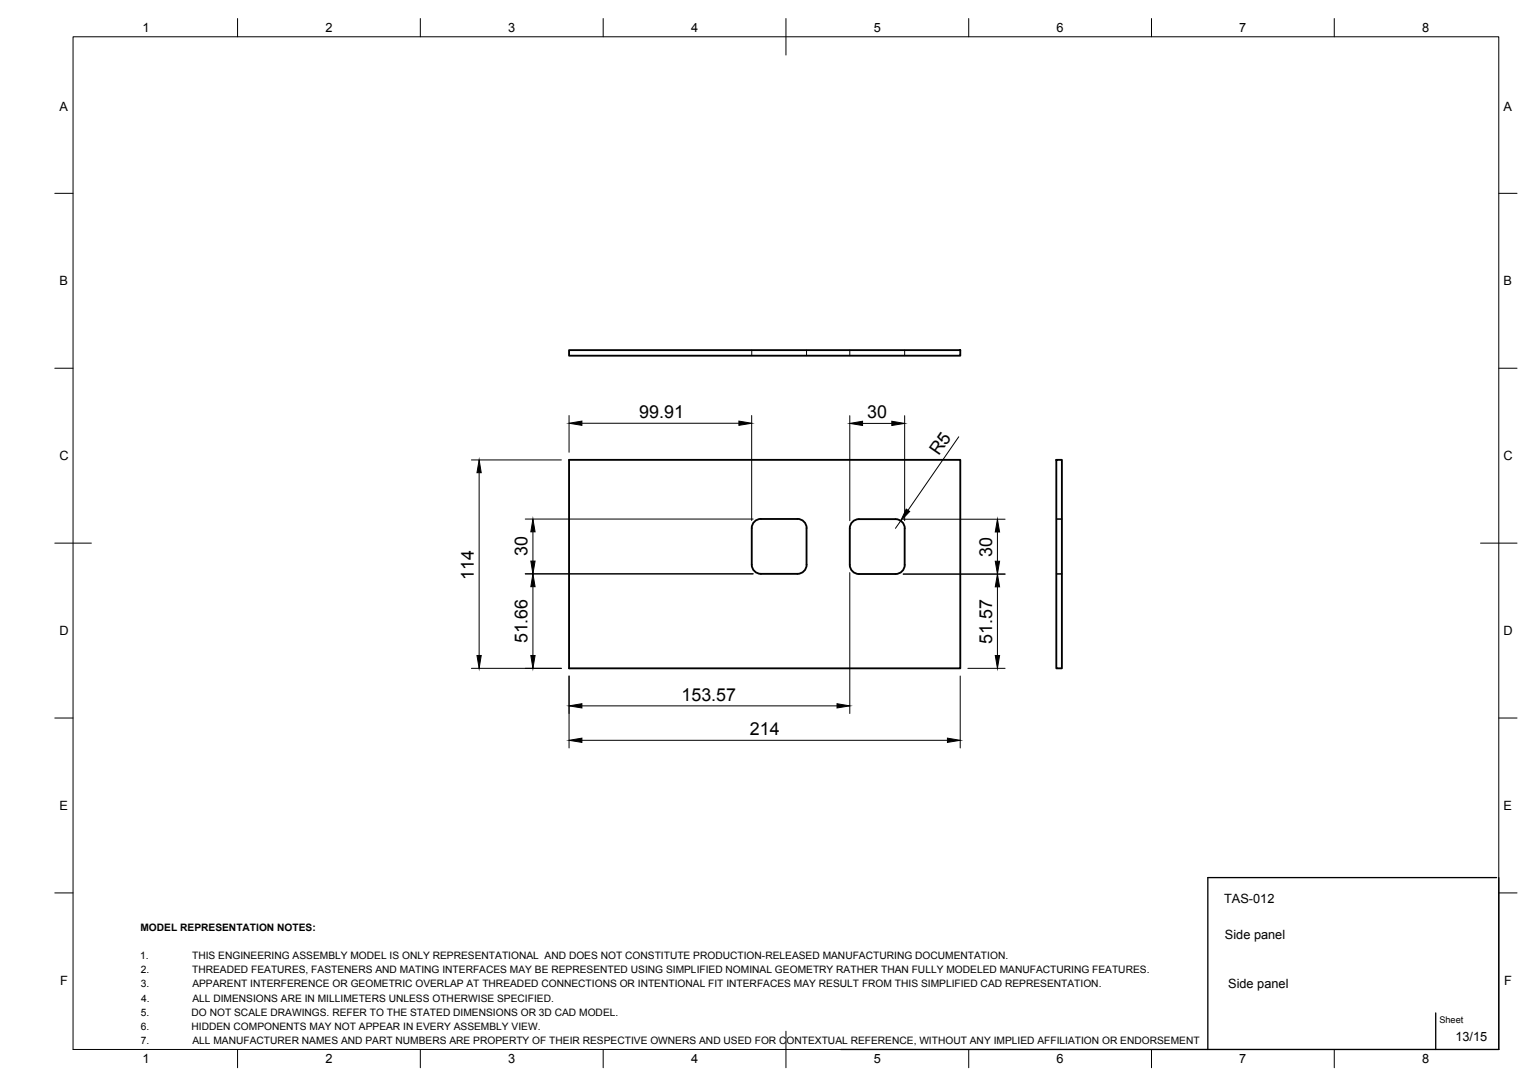
ISO-10303-21;
HEADER;
/* Generated by software containing ST-Developer
 * from STEP Tools, Inc. (www.steptools.com) 
 */

FILE_DESCRIPTION(
/* description */ (
'Independent welded steel electronics enclosure with removable sealed 
lid, internal mounting tray and two threaded cable entries. 300 x 220 
mm body. No ingress or electrical safety rating assigned.'),
/* implementation_level */ '2;1');

FILE_NAME(
/* name */ 'Side panel.step',
/* time_stamp */ '2026-11-14T09:13:27-08:00',
/* author */ (''),
/* organization */ (''),
/* preprocessor_version */ 'ST-DEVELOPER v20.2',
/* originating_system */ 'Autodesk Translation Framework v15.17.0.0',
/* authorisation */ '');

FILE_SCHEMA (('AUTOMOTIVE_DESIGN { 1 0 10303 214 3 1 1 }'));
ENDSEC;

DATA;
#10=MECHANICAL_DESIGN_GEOMETRIC_PRESENTATION_REPRESENTATION('',(#969),#94412);
#939=SHAPE_REPRESENTATION_RELATIONSHIP('SRR','None',#94491,#954);
#954=ADVANCED_BREP_SHAPE_REPRESENTATION('',(#984),#94400);
#969=STYLED_ITEM('',(#94576),#984);
#984=MANIFOLD_SOLID_BREP('Body1',#8254);
#1008=FACE_BOUND('',#1568,.T.);
#1009=FACE_BOUND('',#1569,.T.);
#1010=FACE_BOUND('',#1572,.T.);
#1011=FACE_BOUND('',#1573,.T.);
#1076=PLANE('',#8477);
#1077=PLANE('',#8481);
#1078=PLANE('',#8485);
#1079=PLANE('',#8489);
#1080=PLANE('',#8493);
#1081=PLANE('',#8497);
#1082=PLANE('',#8501);
#1083=PLANE('',#8505);
#1084=PLANE('',#8506);
#1085=PLANE('',#8507);
#1086=PLANE('',#8508);
#1087=PLANE('',#8509);
#1088=PLANE('',#8510);
#1089=PLANE('',#8511);
#1182=FACE_OUTER_BOUND('',#1550,.T.);
#1183=FACE_OUTER_BOUND('',#1551,.T.);
#1184=FACE_OUTER_BOUND('',#1552,.T.);
#1185=FACE_OUTER_BOUND('',#1553,.T.);
#1186=FACE_OUTER_BOUND('',#1554,.T.);
#1187=FACE_OUTER_BOUND('',#1555,.T.);
#1188=FACE_OUTER_BOUND('',#1556,.T.);
#1189=FACE_OUTER_BOUND('',#1557,.T.);
#1190=FACE_OUTER_BOUND('',#1558,.T.);
#1191=FACE_OUTER_BOUND('',#1559,.T.);
#1192=FACE_OUTER_BOUND('',#1560,.T.);
#1193=FACE_OUTER_BOUND('',#1561,.T.);
#1194=FACE_OUTER_BOUND('',#1562,.T.);
#1195=FACE_OUTER_BOUND('',#1563,.T.);
#1196=FACE_OUTER_BOUND('',#1564,.T.);
#1197=FACE_OUTER_BOUND('',#1565,.T.);
#1198=FACE_OUTER_BOUND('',#1566,.T.);
#1199=FACE_OUTER_BOUND('',#1567,.T.);
#1200=FACE_OUTER_BOUND('',#1570,.T.);
#1201=FACE_OUTER_BOUND('',#1571,.T.);
#1202=FACE_OUTER_BOUND('',#1574,.T.);
#1203=FACE_OUTER_BOUND('',#1575,.T.);
#1550=EDGE_LOOP('',(#5202,#5203,#5204,#5205));
#1551=EDGE_LOOP('',(#5206,#5207,#5208,#5209));
#1552=EDGE_LOOP('',(#5210,#5211,#5212,#5213));
#1553=EDGE_LOOP('',(#5214,#5215,#5216,#5217));
#1554=EDGE_LOOP('',(#5218,#5219,#5220,#5221));
#1555=EDGE_LOOP('',(#5222,#5223,#5224,#5225));
#1556=EDGE_LOOP('',(#5226,#5227,#5228,#5229));
#1557=EDGE_LOOP('',(#5230,#5231,#5232,#5233));
#1558=EDGE_LOOP('',(#5234,#5235,#5236,#5237));
#1559=EDGE_LOOP('',(#5238,#5239,#5240,#5241));
#1560=EDGE_LOOP('',(#5242,#5243,#5244,#5245));
#1561=EDGE_LOOP('',(#5246,#5247,#5248,#5249));
#1562=EDGE_LOOP('',(#5250,#5251,#5252,#5253));
#1563=EDGE_LOOP('',(#5254,#5255,#5256,#5257));
#1564=EDGE_LOOP('',(#5258,#5259,#5260,#5261));
#1565=EDGE_LOOP('',(#5262,#5263,#5264,#5265));
#1566=EDGE_LOOP('',(#5266,#5267,#5268,#5269));
#1567=EDGE_LOOP('',(#5270,#5271,#5272,#5273));
#1568=EDGE_LOOP('',(#5274,#5275,#5276,#5277,#5278,#5279,#5280,#5281));
#1569=EDGE_LOOP('',(#5282,#5283,#5284,#5285,#5286,#5287,#5288,#5289));
#1570=EDGE_LOOP('',(#5290,#5291,#5292,#5293));
#1571=EDGE_LOOP('',(#5294,#5295,#5296,#5297));
#1572=EDGE_LOOP('',(#5298,#5299,#5300,#5301,#5302,#5303,#5304,#5305));
#1573=EDGE_LOOP('',(#5306,#5307,#5308,#5309,#5310,#5311,#5312,#5313));
#1574=EDGE_LOOP('',(#5314,#5315,#5316,#5317));
#1575=EDGE_LOOP('',(#5318,#5319,#5320,#5321));
#1974=LINE('',#10485,#2372);
#1975=LINE('',#10488,#2373);
#1976=LINE('',#10491,#2374);
#1977=LINE('',#10493,#2375);
#1978=LINE('',#10494,#2376);
#1979=LINE('',#10499,#2377);
#1980=LINE('',#10503,#2378);
#1981=LINE('',#10505,#2379);
#1982=LINE('',#10506,#2380);
#1983=LINE('',#10512,#2381);
#1984=LINE('',#10515,#2382);
#1985=LINE('',#10517,#2383);
#1986=LINE('',#10518,#2384);
#1987=LINE('',#10523,#2385);
#1988=LINE('',#10526,#2386);
#1989=LINE('',#10527,#2387);
#1990=LINE('',#10533,#2388);
#1991=LINE('',#10536,#2389);
#1992=LINE('',#10539,#2390);
#1993=LINE('',#10541,#2391);
#1994=LINE('',#10542,#2392);
#1995=LINE('',#10548,#2393);
#1996=LINE('',#10551,#2394);
#1997=LINE('',#10553,#2395);
#1998=LINE('',#10554,#2396);
#1999=LINE('',#10559,#2397);
#2000=LINE('',#10563,#2398);
#2001=LINE('',#10565,#2399);
#2002=LINE('',#10566,#2400);
#2003=LINE('',#10571,#2401);
#2004=LINE('',#10574,#2402);
#2005=LINE('',#10575,#2403);
#2006=LINE('',#10579,#2404);
#2007=LINE('',#10581,#2405);
#2008=LINE('',#10583,#2406);
#2009=LINE('',#10584,#2407);
#2010=LINE('',#10587,#2408);
#2011=LINE('',#10589,#2409);
#2012=LINE('',#10590,#2410);
#2013=LINE('',#10593,#2411);
#2014=LINE('',#10595,#2412);
#2015=LINE('',#10596,#2413);
#2016=LINE('',#10598,#2414);
#2017=LINE('',#10599,#2415);
#2372=VECTOR('',#9072,10.);
#2373=VECTOR('',#9075,10.);
#2374=VECTOR('',#9078,10.);
#2375=VECTOR('',#9079,10.);
#2376=VECTOR('',#9080,10.);
#2377=VECTOR('',#9085,10.);
#2378=VECTOR('',#9090,10.);
#2379=VECTOR('',#9091,10.);
#2380=VECTOR('',#9092,10.);
#2381=VECTOR('',#9097,10.);
#2382=VECTOR('',#9100,10.);
#2383=VECTOR('',#9103,10.);
#2384=VECTOR('',#9104,10.);
#2385=VECTOR('',#9109,10.);
#2386=VECTOR('',#9114,10.);
#2387=VECTOR('',#9115,10.);
#2388=VECTOR('',#9120,10.);
#2389=VECTOR('',#9123,10.);
#2390=VECTOR('',#9126,10.);
#2391=VECTOR('',#9127,10.);
#2392=VECTOR('',#9128,10.);
#2393=VECTOR('',#9133,10.);
#2394=VECTOR('',#9136,10.);
#2395=VECTOR('',#9139,10.);
#2396=VECTOR('',#9140,10.);
#2397=VECTOR('',#9145,10.);
#2398=VECTOR('',#9150,10.);
#2399=VECTOR('',#9151,10.);
#2400=VECTOR('',#9152,10.);
#2401=VECTOR('',#9157,10.);
#2402=VECTOR('',#9162,10.);
#2403=VECTOR('',#9163,10.);
#2404=VECTOR('',#9166,10.);
#2405=VECTOR('',#9167,10.);
#2406=VECTOR('',#9168,10.);
#2407=VECTOR('',#9169,10.);
#2408=VECTOR('',#9172,10.);
#2409=VECTOR('',#9173,10.);
#2410=VECTOR('',#9174,10.);
#2411=VECTOR('',#9177,10.);
#2412=VECTOR('',#9178,10.);
#2413=VECTOR('',#9179,10.);
#2414=VECTOR('',#9182,10.);
#2415=VECTOR('',#9183,10.);
#2740=CIRCLE('',#8475,5.);
#2741=CIRCLE('',#8476,5.);
#2742=CIRCLE('',#8479,5.);
#2743=CIRCLE('',#8480,5.);
#2744=CIRCLE('',#8483,5.);
#2745=CIRCLE('',#8484,5.);
#2746=CIRCLE('',#8487,5.);
#2747=CIRCLE('',#8488,5.);
#2748=CIRCLE('',#8491,5.);
#2749=CIRCLE('',#8492,5.);
#2750=CIRCLE('',#8495,5.);
#2751=CIRCLE('',#8496,5.);
#2752=CIRCLE('',#8499,5.);
#2753=CIRCLE('',#8500,5.);
#2754=CIRCLE('',#8503,5.);
#2755=CIRCLE('',#8504,5.);
#2882=VERTEX_POINT('',#10481);
#2883=VERTEX_POINT('',#10482);
#2884=VERTEX_POINT('',#10484);
#2885=VERTEX_POINT('',#10486);
#2886=VERTEX_POINT('',#10490);
#2887=VERTEX_POINT('',#10492);
#2888=VERTEX_POINT('',#10496);
#2889=VERTEX_POINT('',#10498);
#2890=VERTEX_POINT('',#10502);
#2891=VERTEX_POINT('',#10504);
#2892=VERTEX_POINT('',#10508);
#2893=VERTEX_POINT('',#10509);
#2894=VERTEX_POINT('',#10511);
#2895=VERTEX_POINT('',#10513);
#2896=VERTEX_POINT('',#10520);
#2897=VERTEX_POINT('',#10522);
#2898=VERTEX_POINT('',#10529);
#2899=VERTEX_POINT('',#10530);
#2900=VERTEX_POINT('',#10532);
#2901=VERTEX_POINT('',#10534);
#2902=VERTEX_POINT('',#10538);
#2903=VERTEX_POINT('',#10540);
#2904=VERTEX_POINT('',#10544);
#2905=VERTEX_POINT('',#10545);
#2906=VERTEX_POINT('',#10547);
#2907=VERTEX_POINT('',#10549);
#2908=VERTEX_POINT('',#10556);
#2909=VERTEX_POINT('',#10558);
#2910=VERTEX_POINT('',#10562);
#2911=VERTEX_POINT('',#10564);
#2912=VERTEX_POINT('',#10568);
#2913=VERTEX_POINT('',#10570);
#2914=VERTEX_POINT('',#10577);
#2915=VERTEX_POINT('',#10578);
#2916=VERTEX_POINT('',#10580);
#2917=VERTEX_POINT('',#10582);
#2918=VERTEX_POINT('',#10586);
#2919=VERTEX_POINT('',#10588);
#2920=VERTEX_POINT('',#10592);
#2921=VERTEX_POINT('',#10594);
#3866=EDGE_CURVE('',#2882,#2883,#2740,.T.);
#3867=EDGE_CURVE('',#2883,#2884,#1974,.T.);
#3868=EDGE_CURVE('',#2884,#2885,#2741,.T.);
#3869=EDGE_CURVE('',#2885,#2882,#1975,.T.);
#3870=EDGE_CURVE('',#2886,#2883,#1976,.T.);
#3871=EDGE_CURVE('',#2887,#2886,#1977,.T.);
#3872=EDGE_CURVE('',#2884,#2887,#1978,.T.);
#3873=EDGE_CURVE('',#2886,#2888,#2742,.T.);
#3874=EDGE_CURVE('',#2888,#2889,#1979,.T.);
#3875=EDGE_CURVE('',#2889,#2887,#2743,.T.);
#3876=EDGE_CURVE('',#2890,#2888,#1980,.T.);
#3877=EDGE_CURVE('',#2891,#2890,#1981,.T.);
#3878=EDGE_CURVE('',#2889,#2891,#1982,.T.);
#3879=EDGE_CURVE('',#2892,#2893,#2744,.T.);
#3880=EDGE_CURVE('',#2893,#2894,#1983,.T.);
#3881=EDGE_CURVE('',#2894,#2895,#2745,.T.);
#3882=EDGE_CURVE('',#2895,#2892,#1984,.T.);
#3883=EDGE_CURVE('',#2894,#2885,#1985,.T.);
#3884=EDGE_CURVE('',#2882,#2893,#1986,.T.);
#3885=EDGE_CURVE('',#2890,#2896,#2746,.T.);
#3886=EDGE_CURVE('',#2896,#2897,#1987,.T.);
#3887=EDGE_CURVE('',#2897,#2891,#2747,.T.);
#3888=EDGE_CURVE('',#2897,#2895,#1988,.T.);
#3889=EDGE_CURVE('',#2892,#2896,#1989,.T.);
#3890=EDGE_CURVE('',#2898,#2899,#2748,.T.);
#3891=EDGE_CURVE('',#2899,#2900,#1990,.T.);
#3892=EDGE_CURVE('',#2900,#2901,#2749,.T.);
#3893=EDGE_CURVE('',#2901,#2898,#1991,.T.);
#3894=EDGE_CURVE('',#2902,#2899,#1992,.T.);
#3895=EDGE_CURVE('',#2903,#2902,#1993,.T.);
#3896=EDGE_CURVE('',#2900,#2903,#1994,.T.);
#3897=EDGE_CURVE('',#2904,#2905,#2750,.T.);
#3898=EDGE_CURVE('',#2905,#2906,#1995,.T.);
#3899=EDGE_CURVE('',#2906,#2907,#2751,.T.);
#3900=EDGE_CURVE('',#2907,#2904,#1996,.T.);
#3901=EDGE_CURVE('',#2906,#2901,#1997,.T.);
#3902=EDGE_CURVE('',#2898,#2905,#1998,.T.);
#3903=EDGE_CURVE('',#2902,#2908,#2752,.T.);
#3904=EDGE_CURVE('',#2908,#2909,#1999,.T.);
#3905=EDGE_CURVE('',#2909,#2903,#2753,.T.);
#3906=EDGE_CURVE('',#2910,#2908,#2000,.T.);
#3907=EDGE_CURVE('',#2911,#2910,#2001,.T.);
#3908=EDGE_CURVE('',#2909,#2911,#2002,.T.);
#3909=EDGE_CURVE('',#2910,#2912,#2754,.T.);
#3910=EDGE_CURVE('',#2912,#2913,#2003,.T.);
#3911=EDGE_CURVE('',#2913,#2911,#2755,.T.);
#3912=EDGE_CURVE('',#2913,#2907,#2004,.T.);
#3913=EDGE_CURVE('',#2904,#2912,#2005,.T.);
#3914=EDGE_CURVE('',#2914,#2915,#2006,.T.);
#3915=EDGE_CURVE('',#2915,#2916,#2007,.T.);
#3916=EDGE_CURVE('',#2917,#2916,#2008,.T.);
#3917=EDGE_CURVE('',#2914,#2917,#2009,.T.);
#3918=EDGE_CURVE('',#2918,#2914,#2010,.T.);
#3919=EDGE_CURVE('',#2919,#2917,#2011,.T.);
#3920=EDGE_CURVE('',#2918,#2919,#2012,.T.);
#3921=EDGE_CURVE('',#2920,#2918,#2013,.T.);
#3922=EDGE_CURVE('',#2921,#2919,#2014,.T.);
#3923=EDGE_CURVE('',#2920,#2921,#2015,.T.);
#3924=EDGE_CURVE('',#2915,#2920,#2016,.T.);
#3925=EDGE_CURVE('',#2916,#2921,#2017,.T.);
#5202=ORIENTED_EDGE('',*,*,#3866,.T.);
#5203=ORIENTED_EDGE('',*,*,#3867,.T.);
#5204=ORIENTED_EDGE('',*,*,#3868,.T.);
#5205=ORIENTED_EDGE('',*,*,#3869,.T.);
#5206=ORIENTED_EDGE('',*,*,#3867,.F.);
#5207=ORIENTED_EDGE('',*,*,#3870,.F.);
#5208=ORIENTED_EDGE('',*,*,#3871,.F.);
#5209=ORIENTED_EDGE('',*,*,#3872,.F.);
#5210=ORIENTED_EDGE('',*,*,#3873,.T.);
#5211=ORIENTED_EDGE('',*,*,#3874,.T.);
#5212=ORIENTED_EDGE('',*,*,#3875,.T.);
#5213=ORIENTED_EDGE('',*,*,#3871,.T.);
#5214=ORIENTED_EDGE('',*,*,#3874,.F.);
#5215=ORIENTED_EDGE('',*,*,#3876,.F.);
#5216=ORIENTED_EDGE('',*,*,#3877,.F.);
#5217=ORIENTED_EDGE('',*,*,#3878,.F.);
#5218=ORIENTED_EDGE('',*,*,#3879,.T.);
#5219=ORIENTED_EDGE('',*,*,#3880,.T.);
#5220=ORIENTED_EDGE('',*,*,#3881,.T.);
#5221=ORIENTED_EDGE('',*,*,#3882,.T.);
#5222=ORIENTED_EDGE('',*,*,#3869,.F.);
#5223=ORIENTED_EDGE('',*,*,#3883,.F.);
#5224=ORIENTED_EDGE('',*,*,#3880,.F.);
#5225=ORIENTED_EDGE('',*,*,#3884,.F.);
#5226=ORIENTED_EDGE('',*,*,#3885,.T.);
#5227=ORIENTED_EDGE('',*,*,#3886,.T.);
#5228=ORIENTED_EDGE('',*,*,#3887,.T.);
#5229=ORIENTED_EDGE('',*,*,#3877,.T.);
#5230=ORIENTED_EDGE('',*,*,#3882,.F.);
#5231=ORIENTED_EDGE('',*,*,#3888,.F.);
#5232=ORIENTED_EDGE('',*,*,#3886,.F.);
#5233=ORIENTED_EDGE('',*,*,#3889,.F.);
#5234=ORIENTED_EDGE('',*,*,#3890,.T.);
#5235=ORIENTED_EDGE('',*,*,#3891,.T.);
#5236=ORIENTED_EDGE('',*,*,#3892,.T.);
#5237=ORIENTED_EDGE('',*,*,#3893,.T.);
#5238=ORIENTED_EDGE('',*,*,#3891,.F.);
#5239=ORIENTED_EDGE('',*,*,#3894,.F.);
#5240=ORIENTED_EDGE('',*,*,#3895,.F.);
#5241=ORIENTED_EDGE('',*,*,#3896,.F.);
#5242=ORIENTED_EDGE('',*,*,#3897,.T.);
#5243=ORIENTED_EDGE('',*,*,#3898,.T.);
#5244=ORIENTED_EDGE('',*,*,#3899,.T.);
#5245=ORIENTED_EDGE('',*,*,#3900,.T.);
#5246=ORIENTED_EDGE('',*,*,#3893,.F.);
#5247=ORIENTED_EDGE('',*,*,#3901,.F.);
#5248=ORIENTED_EDGE('',*,*,#3898,.F.);
#5249=ORIENTED_EDGE('',*,*,#3902,.F.);
#5250=ORIENTED_EDGE('',*,*,#3903,.T.);
#5251=ORIENTED_EDGE('',*,*,#3904,.T.);
#5252=ORIENTED_EDGE('',*,*,#3905,.T.);
#5253=ORIENTED_EDGE('',*,*,#3895,.T.);
#5254=ORIENTED_EDGE('',*,*,#3904,.F.);
#5255=ORIENTED_EDGE('',*,*,#3906,.F.);
#5256=ORIENTED_EDGE('',*,*,#3907,.F.);
#5257=ORIENTED_EDGE('',*,*,#3908,.F.);
#5258=ORIENTED_EDGE('',*,*,#3909,.T.);
#5259=ORIENTED_EDGE('',*,*,#3910,.T.);
#5260=ORIENTED_EDGE('',*,*,#3911,.T.);
#5261=ORIENTED_EDGE('',*,*,#3907,.T.);
#5262=ORIENTED_EDGE('',*,*,#3900,.F.);
#5263=ORIENTED_EDGE('',*,*,#3912,.F.);
#5264=ORIENTED_EDGE('',*,*,#3910,.F.);
#5265=ORIENTED_EDGE('',*,*,#3913,.F.);
#5266=ORIENTED_EDGE('',*,*,#3914,.T.);
#5267=ORIENTED_EDGE('',*,*,#3915,.T.);
#5268=ORIENTED_EDGE('',*,*,#3916,.F.);
#5269=ORIENTED_EDGE('',*,*,#3917,.F.);
#5270=ORIENTED_EDGE('',*,*,#3918,.T.);
#5271=ORIENTED_EDGE('',*,*,#3917,.T.);
#5272=ORIENTED_EDGE('',*,*,#3919,.F.);
#5273=ORIENTED_EDGE('',*,*,#3920,.F.);
#5274=ORIENTED_EDGE('',*,*,#3906,.T.);
#5275=ORIENTED_EDGE('',*,*,#3903,.F.);
#5276=ORIENTED_EDGE('',*,*,#3894,.T.);
#5277=ORIENTED_EDGE('',*,*,#3890,.F.);
#5278=ORIENTED_EDGE('',*,*,#3902,.T.);
#5279=ORIENTED_EDGE('',*,*,#3897,.F.);
#5280=ORIENTED_EDGE('',*,*,#3913,.T.);
#5281=ORIENTED_EDGE('',*,*,#3909,.F.);
#5282=ORIENTED_EDGE('',*,*,#3870,.T.);
#5283=ORIENTED_EDGE('',*,*,#3866,.F.);
#5284=ORIENTED_EDGE('',*,*,#3884,.T.);
#5285=ORIENTED_EDGE('',*,*,#3879,.F.);
#5286=ORIENTED_EDGE('',*,*,#3889,.T.);
#5287=ORIENTED_EDGE('',*,*,#3885,.F.);
#5288=ORIENTED_EDGE('',*,*,#3876,.T.);
#5289=ORIENTED_EDGE('',*,*,#3873,.F.);
#5290=ORIENTED_EDGE('',*,*,#3921,.T.);
#5291=ORIENTED_EDGE('',*,*,#3920,.T.);
#5292=ORIENTED_EDGE('',*,*,#3922,.F.);
#5293=ORIENTED_EDGE('',*,*,#3923,.F.);
#5294=ORIENTED_EDGE('',*,*,#3924,.T.);
#5295=ORIENTED_EDGE('',*,*,#3923,.T.);
#5296=ORIENTED_EDGE('',*,*,#3925,.F.);
#5297=ORIENTED_EDGE('',*,*,#3915,.F.);
#5298=ORIENTED_EDGE('',*,*,#3908,.T.);
#5299=ORIENTED_EDGE('',*,*,#3911,.F.);
#5300=ORIENTED_EDGE('',*,*,#3912,.T.);
#5301=ORIENTED_EDGE('',*,*,#3899,.F.);
#5302=ORIENTED_EDGE('',*,*,#3901,.T.);
#5303=ORIENTED_EDGE('',*,*,#3892,.F.);
#5304=ORIENTED_EDGE('',*,*,#3896,.T.);
#5305=ORIENTED_EDGE('',*,*,#3905,.F.);
#5306=ORIENTED_EDGE('',*,*,#3872,.T.);
#5307=ORIENTED_EDGE('',*,*,#3875,.F.);
#5308=ORIENTED_EDGE('',*,*,#3878,.T.);
#5309=ORIENTED_EDGE('',*,*,#3887,.F.);
#5310=ORIENTED_EDGE('',*,*,#3888,.T.);
#5311=ORIENTED_EDGE('',*,*,#3881,.F.);
#5312=ORIENTED_EDGE('',*,*,#3883,.T.);
#5313=ORIENTED_EDGE('',*,*,#3868,.F.);
#5314=ORIENTED_EDGE('',*,*,#3925,.T.);
#5315=ORIENTED_EDGE('',*,*,#3922,.T.);
#5316=ORIENTED_EDGE('',*,*,#3919,.T.);
#5317=ORIENTED_EDGE('',*,*,#3916,.T.);
#5318=ORIENTED_EDGE('',*,*,#3924,.F.);
#5319=ORIENTED_EDGE('',*,*,#3914,.F.);
#5320=ORIENTED_EDGE('',*,*,#3918,.F.);
#5321=ORIENTED_EDGE('',*,*,#3921,.F.);
#7664=CYLINDRICAL_SURFACE('',#8474,5.);
#7665=CYLINDRICAL_SURFACE('',#8478,5.);
#7666=CYLINDRICAL_SURFACE('',#8482,5.);
#7667=CYLINDRICAL_SURFACE('',#8486,5.);
#7668=CYLINDRICAL_SURFACE('',#8490,5.);
#7669=CYLINDRICAL_SURFACE('',#8494,5.);
#7670=CYLINDRICAL_SURFACE('',#8498,5.);
#7671=CYLINDRICAL_SURFACE('',#8502,5.);
#7919=ADVANCED_FACE('',(#1182),#7664,.F.);
#7920=ADVANCED_FACE('',(#1183),#1076,.F.);
#7921=ADVANCED_FACE('',(#1184),#7665,.F.);
#7922=ADVANCED_FACE('',(#1185),#1077,.F.);
#7923=ADVANCED_FACE('',(#1186),#7666,.F.);
#7924=ADVANCED_FACE('',(#1187),#1078,.F.);
#7925=ADVANCED_FACE('',(#1188),#7667,.F.);
#7926=ADVANCED_FACE('',(#1189),#1079,.F.);
#7927=ADVANCED_FACE('',(#1190),#7668,.F.);
#7928=ADVANCED_FACE('',(#1191),#1080,.F.);
#7929=ADVANCED_FACE('',(#1192),#7669,.F.);
#7930=ADVANCED_FACE('',(#1193),#1081,.F.);
#7931=ADVANCED_FACE('',(#1194),#7670,.F.);
#7932=ADVANCED_FACE('',(#1195),#1082,.F.);
#7933=ADVANCED_FACE('',(#1196),#7671,.F.);
#7934=ADVANCED_FACE('',(#1197),#1083,.F.);
#7935=ADVANCED_FACE('',(#1198),#1084,.T.);
#7936=ADVANCED_FACE('',(#1199,#1008,#1009),#1085,.T.);
#7937=ADVANCED_FACE('',(#1200),#1086,.T.);
#7938=ADVANCED_FACE('',(#1201,#1010,#1011),#1087,.T.);
#7939=ADVANCED_FACE('',(#1202),#1088,.T.);
#7940=ADVANCED_FACE('',(#1203),#1089,.F.);
#8254=CLOSED_SHELL('',(#7919,#7920,#7921,#7922,#7923,#7924,#7925,#7926,
#7927,#7928,#7929,#7930,#7931,#7932,#7933,#7934,#7935,#7936,#7937,#7938,
#7939,#7940));
#8473=AXIS2_PLACEMENT_3D('',#10479,#9066,#9067);
#8474=AXIS2_PLACEMENT_3D('',#10480,#9068,#9069);
#8475=AXIS2_PLACEMENT_3D('',#10483,#9070,#9071);
#8476=AXIS2_PLACEMENT_3D('',#10487,#9073,#9074);
#8477=AXIS2_PLACEMENT_3D('',#10489,#9076,#9077);
#8478=AXIS2_PLACEMENT_3D('',#10495,#9081,#9082);
#8479=AXIS2_PLACEMENT_3D('',#10497,#9083,#9084);
#8480=AXIS2_PLACEMENT_3D('',#10500,#9086,#9087);
#8481=AXIS2_PLACEMENT_3D('',#10501,#9088,#9089);
#8482=AXIS2_PLACEMENT_3D('',#10507,#9093,#9094);
#8483=AXIS2_PLACEMENT_3D('',#10510,#9095,#9096);
#8484=AXIS2_PLACEMENT_3D('',#10514,#9098,#9099);
#8485=AXIS2_PLACEMENT_3D('',#10516,#9101,#9102);
#8486=AXIS2_PLACEMENT_3D('',#10519,#9105,#9106);
#8487=AXIS2_PLACEMENT_3D('',#10521,#9107,#9108);
#8488=AXIS2_PLACEMENT_3D('',#10524,#9110,#9111);
#8489=AXIS2_PLACEMENT_3D('',#10525,#9112,#9113);
#8490=AXIS2_PLACEMENT_3D('',#10528,#9116,#9117);
#8491=AXIS2_PLACEMENT_3D('',#10531,#9118,#9119);
#8492=AXIS2_PLACEMENT_3D('',#10535,#9121,#9122);
#8493=AXIS2_PLACEMENT_3D('',#10537,#9124,#9125);
#8494=AXIS2_PLACEMENT_3D('',#10543,#9129,#9130);
#8495=AXIS2_PLACEMENT_3D('',#10546,#9131,#9132);
#8496=AXIS2_PLACEMENT_3D('',#10550,#9134,#9135);
#8497=AXIS2_PLACEMENT_3D('',#10552,#9137,#9138);
#8498=AXIS2_PLACEMENT_3D('',#10555,#9141,#9142);
#8499=AXIS2_PLACEMENT_3D('',#10557,#9143,#9144);
#8500=AXIS2_PLACEMENT_3D('',#10560,#9146,#9147);
#8501=AXIS2_PLACEMENT_3D('',#10561,#9148,#9149);
#8502=AXIS2_PLACEMENT_3D('',#10567,#9153,#9154);
#8503=AXIS2_PLACEMENT_3D('',#10569,#9155,#9156);
#8504=AXIS2_PLACEMENT_3D('',#10572,#9158,#9159);
#8505=AXIS2_PLACEMENT_3D('',#10573,#9160,#9161);
#8506=AXIS2_PLACEMENT_3D('',#10576,#9164,#9165);
#8507=AXIS2_PLACEMENT_3D('',#10585,#9170,#9171);
#8508=AXIS2_PLACEMENT_3D('',#10591,#9175,#9176);
#8509=AXIS2_PLACEMENT_3D('',#10597,#9180,#9181);
#8510=AXIS2_PLACEMENT_3D('',#10600,#9184,#9185);
#8511=AXIS2_PLACEMENT_3D('',#10601,#9186,#9187);
#9066=DIRECTION('axis',(0.,0.,1.));
#9067=DIRECTION('refdir',(1.,0.,0.));
#9068=DIRECTION('center_axis',(-1.,0.,0.));
#9069=DIRECTION('ref_axis',(0.,-0.707106781186548,0.707106781186548));
#9070=DIRECTION('center_axis',(1.,0.,0.));
#9071=DIRECTION('ref_axis',(0.,-0.707106781186548,0.707106781186548));
#9072=DIRECTION('',(-1.,0.,0.));
#9073=DIRECTION('center_axis',(-1.,0.,0.));
#9074=DIRECTION('ref_axis',(0.,-0.707106781186548,0.707106781186548));
#9075=DIRECTION('',(1.,0.,0.));
#9076=DIRECTION('center_axis',(0.,-1.,0.));
#9077=DIRECTION('ref_axis',(0.,0.,1.));
#9078=DIRECTION('',(0.,0.,1.));
#9079=DIRECTION('',(1.,0.,0.));
#9080=DIRECTION('',(0.,0.,-1.));
#9081=DIRECTION('center_axis',(-1.,0.,0.));
#9082=DIRECTION('ref_axis',(0.,-0.707106781186548,-0.707106781186548));
#9083=DIRECTION('center_axis',(1.,0.,0.));
#9084=DIRECTION('ref_axis',(0.,-0.707106781186548,-0.707106781186548));
#9085=DIRECTION('',(-1.,0.,0.));
#9086=DIRECTION('center_axis',(-1.,0.,0.));
#9087=DIRECTION('ref_axis',(0.,-0.707106781186548,-0.707106781186548));
#9088=DIRECTION('center_axis',(0.,0.,-1.));
#9089=DIRECTION('ref_axis',(0.,-1.,0.));
#9090=DIRECTION('',(0.,-1.,0.));
#9091=DIRECTION('',(1.,0.,0.));
#9092=DIRECTION('',(0.,1.,0.));
#9093=DIRECTION('center_axis',(-1.,0.,0.));
#9094=DIRECTION('ref_axis',(0.,0.707106781186548,0.707106781186548));
#9095=DIRECTION('center_axis',(1.,0.,0.));
#9096=DIRECTION('ref_axis',(0.,0.707106781186548,0.707106781186548));
#9097=DIRECTION('',(-1.,0.,0.));
#9098=DIRECTION('center_axis',(-1.,0.,0.));
#9099=DIRECTION('ref_axis',(0.,0.707106781186548,0.707106781186548));
#9100=DIRECTION('',(1.,0.,0.));
#9101=DIRECTION('center_axis',(0.,0.,1.));
#9102=DIRECTION('ref_axis',(0.,1.,0.));
#9103=DIRECTION('',(0.,-1.,0.));
#9104=DIRECTION('',(0.,1.,0.));
#9105=DIRECTION('center_axis',(-1.,0.,0.));
#9106=DIRECTION('ref_axis',(0.,0.707106781186548,-0.707106781186548));
#9107=DIRECTION('center_axis',(1.,0.,0.));
#9108=DIRECTION('ref_axis',(0.,0.707106781186548,-0.707106781186548));
#9109=DIRECTION('',(-1.,0.,0.));
#9110=DIRECTION('center_axis',(-1.,0.,0.));
#9111=DIRECTION('ref_axis',(0.,0.707106781186548,-0.707106781186548));
#9112=DIRECTION('center_axis',(0.,1.,0.));
#9113=DIRECTION('ref_axis',(0.,0.,-1.));
#9114=DIRECTION('',(0.,0.,1.));
#9115=DIRECTION('',(0.,0.,-1.));
#9116=DIRECTION('center_axis',(-1.,0.,0.));
#9117=DIRECTION('ref_axis',(0.,0.707106781186548,0.707106781186548));
#9118=DIRECTION('center_axis',(1.,0.,0.));
#9119=DIRECTION('ref_axis',(0.,0.707106781186548,0.707106781186548));
#9120=DIRECTION('',(-1.,0.,0.));
#9121=DIRECTION('center_axis',(-1.,0.,0.));
#9122=DIRECTION('ref_axis',(0.,0.707106781186548,0.707106781186548));
#9123=DIRECTION('',(1.,0.,0.));
#9124=DIRECTION('center_axis',(0.,0.,1.));
#9125=DIRECTION('ref_axis',(0.,1.,0.));
#9126=DIRECTION('',(0.,1.,0.));
#9127=DIRECTION('',(1.,0.,0.));
#9128=DIRECTION('',(0.,-1.,0.));
#9129=DIRECTION('center_axis',(-1.,0.,0.));
#9130=DIRECTION('ref_axis',(0.,0.707106781186548,-0.707106781186548));
#9131=DIRECTION('center_axis',(1.,0.,0.));
#9132=DIRECTION('ref_axis',(0.,0.707106781186548,-0.707106781186548));
#9133=DIRECTION('',(-1.,0.,0.));
#9134=DIRECTION('center_axis',(-1.,0.,0.));
#9135=DIRECTION('ref_axis',(0.,0.707106781186548,-0.707106781186548));
#9136=DIRECTION('',(1.,0.,0.));
#9137=DIRECTION('center_axis',(0.,1.,0.));
#9138=DIRECTION('ref_axis',(0.,0.,-1.));
#9139=DIRECTION('',(0.,0.,1.));
#9140=DIRECTION('',(0.,0.,-1.));
#9141=DIRECTION('center_axis',(-1.,0.,0.));
#9142=DIRECTION('ref_axis',(0.,-0.707106781186548,0.707106781186548));
#9143=DIRECTION('center_axis',(1.,0.,0.));
#9144=DIRECTION('ref_axis',(0.,-0.707106781186548,0.707106781186548));
#9145=DIRECTION('',(-1.,0.,0.));
#9146=DIRECTION('center_axis',(-1.,0.,0.));
#9147=DIRECTION('ref_axis',(0.,-0.707106781186548,0.707106781186548));
#9148=DIRECTION('center_axis',(0.,-1.,0.));
#9149=DIRECTION('ref_axis',(0.,0.,1.));
#9150=DIRECTION('',(0.,0.,1.));
#9151=DIRECTION('',(1.,0.,0.));
#9152=DIRECTION('',(0.,0.,-1.));
#9153=DIRECTION('center_axis',(-1.,0.,0.));
#9154=DIRECTION('ref_axis',(0.,-0.707106781186548,-0.707106781186548));
#9155=DIRECTION('center_axis',(1.,0.,0.));
#9156=DIRECTION('ref_axis',(0.,-0.707106781186548,-0.707106781186548));
#9157=DIRECTION('',(-1.,0.,0.));
#9158=DIRECTION('center_axis',(-1.,0.,0.));
#9159=DIRECTION('ref_axis',(0.,-0.707106781186548,-0.707106781186548));
#9160=DIRECTION('center_axis',(0.,0.,-1.));
#9161=DIRECTION('ref_axis',(0.,-1.,0.));
#9162=DIRECTION('',(0.,1.,0.));
#9163=DIRECTION('',(0.,-1.,0.));
#9164=DIRECTION('center_axis',(0.,1.,0.));
#9165=DIRECTION('ref_axis',(-1.,0.,0.));
#9166=DIRECTION('',(-1.,0.,0.));
#9167=DIRECTION('',(0.,0.,1.));
#9168=DIRECTION('',(-1.,0.,0.));
#9169=DIRECTION('',(0.,0.,1.));
#9170=DIRECTION('center_axis',(1.,0.,0.));
#9171=DIRECTION('ref_axis',(0.,1.,0.));
#9172=DIRECTION('',(0.,1.,0.));
#9173=DIRECTION('',(0.,1.,0.));
#9174=DIRECTION('',(0.,0.,1.));
#9175=DIRECTION('center_axis',(0.,-1.,0.));
#9176=DIRECTION('ref_axis',(1.,0.,0.));
#9177=DIRECTION('',(1.,0.,0.));
#9178=DIRECTION('',(1.,0.,0.));
#9179=DIRECTION('',(0.,0.,1.));
#9180=DIRECTION('center_axis',(-1.,0.,0.));
#9181=DIRECTION('ref_axis',(0.,-1.,0.));
#9182=DIRECTION('',(0.,-1.,0.));
#9183=DIRECTION('',(0.,-1.,0.));
#9184=DIRECTION('center_axis',(0.,0.,1.));
#9185=DIRECTION('ref_axis',(1.,0.,0.));
#9186=DIRECTION('center_axis',(0.,0.,1.));
#9187=DIRECTION('ref_axis',(1.,0.,0.));
#10479=CARTESIAN_POINT('',(0.,0.,0.));
#10480=CARTESIAN_POINT('Origin',(298.5,-17.9108928257202,76.6590099406496));
#10481=CARTESIAN_POINT('',(1.5,-17.9108928257202,81.6590099406496));
#10482=CARTESIAN_POINT('',(1.5,-22.9108928257202,76.6590099406496));
#10483=CARTESIAN_POINT('Origin',(1.49999999999999,-17.9108928257202,76.6590099406496));
#10484=CARTESIAN_POINT('',(-1.5,-22.9108928257202,76.6590099406496));
#10485=CARTESIAN_POINT('',(298.5,-22.9108928257202,76.6590099406496));
#10486=CARTESIAN_POINT('',(-1.5,-17.9108928257202,81.6590099406496));
#10487=CARTESIAN_POINT('Origin',(-1.49999999999999,-17.9108928257202,76.6590099406496));
#10488=CARTESIAN_POINT('',(298.5,-17.9108928257202,81.6590099406496));
#10489=CARTESIAN_POINT('Origin',(298.5,-22.9108928257202,51.6590099406496));
#10490=CARTESIAN_POINT('',(1.5,-22.9108928257202,56.6590099406496));
#10491=CARTESIAN_POINT('',(1.5,-22.9108928257202,25.8295049703248));
#10492=CARTESIAN_POINT('',(-1.5,-22.9108928257202,56.6590099406496));
#10493=CARTESIAN_POINT('',(298.5,-22.9108928257202,56.6590099406496));
#10494=CARTESIAN_POINT('',(-1.5,-22.9108928257202,25.8295049703248));
#10495=CARTESIAN_POINT('Origin',(298.5,-17.9108928257202,56.6590099406496));
#10496=CARTESIAN_POINT('',(1.5,-17.9108928257202,51.6590099406496));
#10497=CARTESIAN_POINT('Origin',(1.49999999999999,-17.9108928257202,56.6590099406496));
#10498=CARTESIAN_POINT('',(-1.5,-17.9108928257202,51.6590099406496));
#10499=CARTESIAN_POINT('',(298.5,-17.9108928257202,51.6590099406496));
#10500=CARTESIAN_POINT('Origin',(-1.49999999999999,-17.9108928257202,56.6590099406496));
#10501=CARTESIAN_POINT('Origin',(298.5,7.0891071742798,51.6590099406496));
#10502=CARTESIAN_POINT('',(1.5,2.0891071742798,51.6590099406496));
#10503=CARTESIAN_POINT('',(1.5,-49.9554464128601,51.6590099406496));
#10504=CARTESIAN_POINT('',(-1.5,2.0891071742798,51.6590099406496));
#10505=CARTESIAN_POINT('',(298.5,2.0891071742798,51.6590099406496));
#10506=CARTESIAN_POINT('',(-1.5,57.0445535871399,51.6590099406496));
#10507=CARTESIAN_POINT('Origin',(298.5,2.0891071742798,76.6590099406496));
#10508=CARTESIAN_POINT('',(1.5,7.0891071742798,76.6590099406496));
#10509=CARTESIAN_POINT('',(1.5,2.0891071742798,81.6590099406496));
#10510=CARTESIAN_POINT('Origin',(1.49999999999999,2.0891071742798,76.6590099406496));
#10511=CARTESIAN_POINT('',(-1.5,2.0891071742798,81.6590099406496));
#10512=CARTESIAN_POINT('',(298.5,2.0891071742798,81.6590099406496));
#10513=CARTESIAN_POINT('',(-1.5,7.0891071742798,76.6590099406496));
#10514=CARTESIAN_POINT('Origin',(-1.49999999999999,2.0891071742798,76.6590099406496));
#10515=CARTESIAN_POINT('',(298.5,7.0891071742798,76.6590099406496));
#10516=CARTESIAN_POINT('Origin',(298.5,-22.9108928257202,81.6590099406496));
#10517=CARTESIAN_POINT('',(-1.5,42.0445535871399,81.6590099406496));
#10518=CARTESIAN_POINT('',(1.5,-64.9554464128601,81.6590099406496));
#10519=CARTESIAN_POINT('Origin',(298.5,2.0891071742798,56.6590099406496));
#10520=CARTESIAN_POINT('',(1.5,7.0891071742798,56.6590099406496));
#10521=CARTESIAN_POINT('Origin',(1.49999999999999,2.0891071742798,56.6590099406496));
#10522=CARTESIAN_POINT('',(-1.5,7.0891071742798,56.6590099406496));
#10523=CARTESIAN_POINT('',(298.5,7.0891071742798,56.6590099406496));
#10524=CARTESIAN_POINT('Origin',(-1.49999999999999,2.0891071742798,56.6590099406496));
#10525=CARTESIAN_POINT('Origin',(298.5,7.0891071742798,81.6590099406496));
#10526=CARTESIAN_POINT('',(-1.5,7.0891071742798,40.8295049703248));
#10527=CARTESIAN_POINT('',(1.5,7.0891071742798,40.8295049703248));
#10528=CARTESIAN_POINT('Origin',(298.5,-51.5734387277091,76.5706645852841));
#10529=CARTESIAN_POINT('',(1.5,-46.5734387277091,76.5706645852841));
#10530=CARTESIAN_POINT('',(1.5,-51.5734387277091,81.5706645852841));
#10531=CARTESIAN_POINT('Origin',(1.49999999999999,-51.5734387277091,76.5706645852841));
#10532=CARTESIAN_POINT('',(-1.5,-51.5734387277091,81.5706645852841));
#10533=CARTESIAN_POINT('',(298.5,-51.5734387277091,81.5706645852841));
#10534=CARTESIAN_POINT('',(-1.5,-46.5734387277091,76.5706645852841));
#10535=CARTESIAN_POINT('Origin',(-1.49999999999999,-51.5734387277091,76.5706645852841));
#10536=CARTESIAN_POINT('',(298.5,-46.5734387277091,76.5706645852841));
#10537=CARTESIAN_POINT('Origin',(298.5,-76.5734387277091,81.5706645852841));
#10538=CARTESIAN_POINT('',(1.5,-71.5734387277091,81.5706645852841));
#10539=CARTESIAN_POINT('',(1.5,-91.7867193638546,81.5706645852841));
#10540=CARTESIAN_POINT('',(-1.5,-71.5734387277091,81.5706645852841));
#10541=CARTESIAN_POINT('',(298.5,-71.5734387277091,81.5706645852841));
#10542=CARTESIAN_POINT('',(-1.5,15.2132806361454,81.5706645852841));
#10543=CARTESIAN_POINT('Origin',(298.5,-51.5734387277091,56.5706645852841));
#10544=CARTESIAN_POINT('',(1.5,-51.5734387277091,51.5706645852841));
#10545=CARTESIAN_POINT('',(1.5,-46.5734387277091,56.5706645852841));
#10546=CARTESIAN_POINT('Origin',(1.49999999999999,-51.5734387277091,56.5706645852841));
#10547=CARTESIAN_POINT('',(-1.5,-46.5734387277091,56.5706645852841));
#10548=CARTESIAN_POINT('',(298.5,-46.5734387277091,56.5706645852841));
#10549=CARTESIAN_POINT('',(-1.5,-51.5734387277091,51.5706645852841));
#10550=CARTESIAN_POINT('Origin',(-1.49999999999999,-51.5734387277091,56.5706645852841));
#10551=CARTESIAN_POINT('',(298.5,-51.5734387277091,51.5706645852841));
#10552=CARTESIAN_POINT('Origin',(298.5,-46.5734387277091,81.5706645852841));
#10553=CARTESIAN_POINT('',(-1.5,-46.5734387277091,40.785332292642));
#10554=CARTESIAN_POINT('',(1.5,-46.5734387277091,40.785332292642));
#10555=CARTESIAN_POINT('Origin',(298.5,-71.5734387277091,76.5706645852841));
#10556=CARTESIAN_POINT('',(1.5,-76.5734387277091,76.5706645852841));
#10557=CARTESIAN_POINT('Origin',(1.49999999999999,-71.5734387277091,76.5706645852841));
#10558=CARTESIAN_POINT('',(-1.5,-76.5734387277091,76.5706645852841));
#10559=CARTESIAN_POINT('',(298.5,-76.5734387277091,76.5706645852841));
#10560=CARTESIAN_POINT('Origin',(-1.49999999999999,-71.5734387277091,76.5706645852841));
#10561=CARTESIAN_POINT('Origin',(298.5,-76.5734387277091,51.5706645852841));
#10562=CARTESIAN_POINT('',(1.5,-76.5734387277091,56.5706645852841));
#10563=CARTESIAN_POINT('',(1.5,-76.5734387277091,25.785332292642));
#10564=CARTESIAN_POINT('',(-1.5,-76.5734387277091,56.5706645852841));
#10565=CARTESIAN_POINT('',(298.5,-76.5734387277091,56.5706645852841));
#10566=CARTESIAN_POINT('',(-1.5,-76.5734387277091,25.785332292642));
#10567=CARTESIAN_POINT('Origin',(298.5,-71.5734387277091,56.5706645852841));
#10568=CARTESIAN_POINT('',(1.5,-71.5734387277091,51.5706645852841));
#10569=CARTESIAN_POINT('Origin',(1.49999999999999,-71.5734387277091,56.5706645852841));
#10570=CARTESIAN_POINT('',(-1.5,-71.5734387277091,51.5706645852841));
#10571=CARTESIAN_POINT('',(298.5,-71.5734387277091,51.5706645852841));
#10572=CARTESIAN_POINT('Origin',(-1.49999999999999,-71.5734387277091,56.5706645852841));
#10573=CARTESIAN_POINT('Origin',(298.5,-46.5734387277091,51.5706645852841));
#10574=CARTESIAN_POINT('',(-1.5,30.2132806361454,51.5706645852841));
#10575=CARTESIAN_POINT('',(1.5,-76.7867193638546,51.5706645852841));
#10576=CARTESIAN_POINT('Origin',(1.5,107.,0.));
#10577=CARTESIAN_POINT('',(1.5,107.,0.));
#10578=CARTESIAN_POINT('',(-1.5,107.,0.));
#10579=CARTESIAN_POINT('',(1.5,107.,0.));
#10580=CARTESIAN_POINT('',(-1.5,107.,114.));
#10581=CARTESIAN_POINT('',(-1.5,107.,0.));
#10582=CARTESIAN_POINT('',(1.5,107.,114.));
#10583=CARTESIAN_POINT('',(1.5,107.,114.));
#10584=CARTESIAN_POINT('',(1.5,107.,0.));
#10585=CARTESIAN_POINT('Origin',(1.5,-107.,0.));
#10586=CARTESIAN_POINT('',(1.5,-107.,0.));
#10587=CARTESIAN_POINT('',(1.5,-107.,0.));
#10588=CARTESIAN_POINT('',(1.5,-107.,114.));
#10589=CARTESIAN_POINT('',(1.5,-107.,114.));
#10590=CARTESIAN_POINT('',(1.5,-107.,0.));
#10591=CARTESIAN_POINT('Origin',(-1.5,-107.,0.));
#10592=CARTESIAN_POINT('',(-1.5,-107.,0.));
#10593=CARTESIAN_POINT('',(-1.5,-107.,0.));
#10594=CARTESIAN_POINT('',(-1.5,-107.,114.));
#10595=CARTESIAN_POINT('',(-1.5,-107.,114.));
#10596=CARTESIAN_POINT('',(-1.5,-107.,0.));
#10597=CARTESIAN_POINT('Origin',(-1.5,107.,0.));
#10598=CARTESIAN_POINT('',(-1.5,107.,0.));
#10599=CARTESIAN_POINT('',(-1.5,107.,114.));
#10600=CARTESIAN_POINT('Origin',(0.,0.,114.));
#10601=CARTESIAN_POINT('Origin',(0.,0.,0.));
#94382=UNCERTAINTY_MEASURE_WITH_UNIT(LENGTH_MEASURE(0.01),#94413,
'DISTANCE_ACCURACY_VALUE',
'Maximum model space distance between geometric entities at asserted c
onnectivities');
#94394=UNCERTAINTY_MEASURE_WITH_UNIT(LENGTH_MEASURE(0.01),#94413,
'DISTANCE_ACCURACY_VALUE',
'Maximum model space distance between geometric entities at asserted c
onnectivities');
#94400=(
GEOMETRIC_REPRESENTATION_CONTEXT(3)
GLOBAL_UNCERTAINTY_ASSIGNED_CONTEXT((#94382))
GLOBAL_UNIT_ASSIGNED_CONTEXT((#94413,#94415,#94416))
REPRESENTATION_CONTEXT('','3D')
);
#94412=(
GEOMETRIC_REPRESENTATION_CONTEXT(3)
GLOBAL_UNCERTAINTY_ASSIGNED_CONTEXT((#94394))
GLOBAL_UNIT_ASSIGNED_CONTEXT((#94413,#94415,#94416))
REPRESENTATION_CONTEXT('','3D')
);
#94413=(
LENGTH_UNIT()
NAMED_UNIT(*)
SI_UNIT(.MILLI.,.METRE.)
);
#94415=(
NAMED_UNIT(*)
PLANE_ANGLE_UNIT()
SI_UNIT($,.RADIAN.)
);
#94416=(
NAMED_UNIT(*)
SI_UNIT($,.STERADIAN.)
SOLID_ANGLE_UNIT()
);
#94422=SHAPE_DEFINITION_REPRESENTATION(#94439,#94491);
#94439=PRODUCT_DEFINITION_SHAPE('',$,#94509);
#94491=SHAPE_REPRESENTATION('',(#8473),#94400);
#94503=PRODUCT_DEFINITION_CONTEXT('part definition',#94556,'design');
#94509=PRODUCT_DEFINITION('Side panel','Side panel',#94526,#94503);
#94526=PRODUCT_DEFINITION_FORMATION('',$,#94563);
#94556=APPLICATION_CONTEXT(
'Core Data for Automotive Mechanical Design Process');
#94557=PRODUCT_CONTEXT('part definition',#94556,'mechanical');
#94563=PRODUCT('Side panel','Side panel',
'3 mm steel sheet; weld adjoining shell-panel edges continuously. Fabr
ication weld specification remains to be selected.',(#94557));
#94576=PRESENTATION_STYLE_ASSIGNMENT((#94583));
#94583=SURFACE_STYLE_USAGE(.BOTH.,#94590);
#94590=SURFACE_SIDE_STYLE('',(#94597));
#94597=SURFACE_STYLE_FILL_AREA(#94604);
#94604=FILL_AREA_STYLE('Opaque(23,69,131)',(#94611));
#94611=FILL_AREA_STYLE_COLOUR('Opaque(23,69,131)',#94618);
#94618=COLOUR_RGB('Opaque(23,69,131)',0.0901960784313725,0.270588235294118,
0.513725490196078);
ENDSEC;
END-ISO-10303-21;
